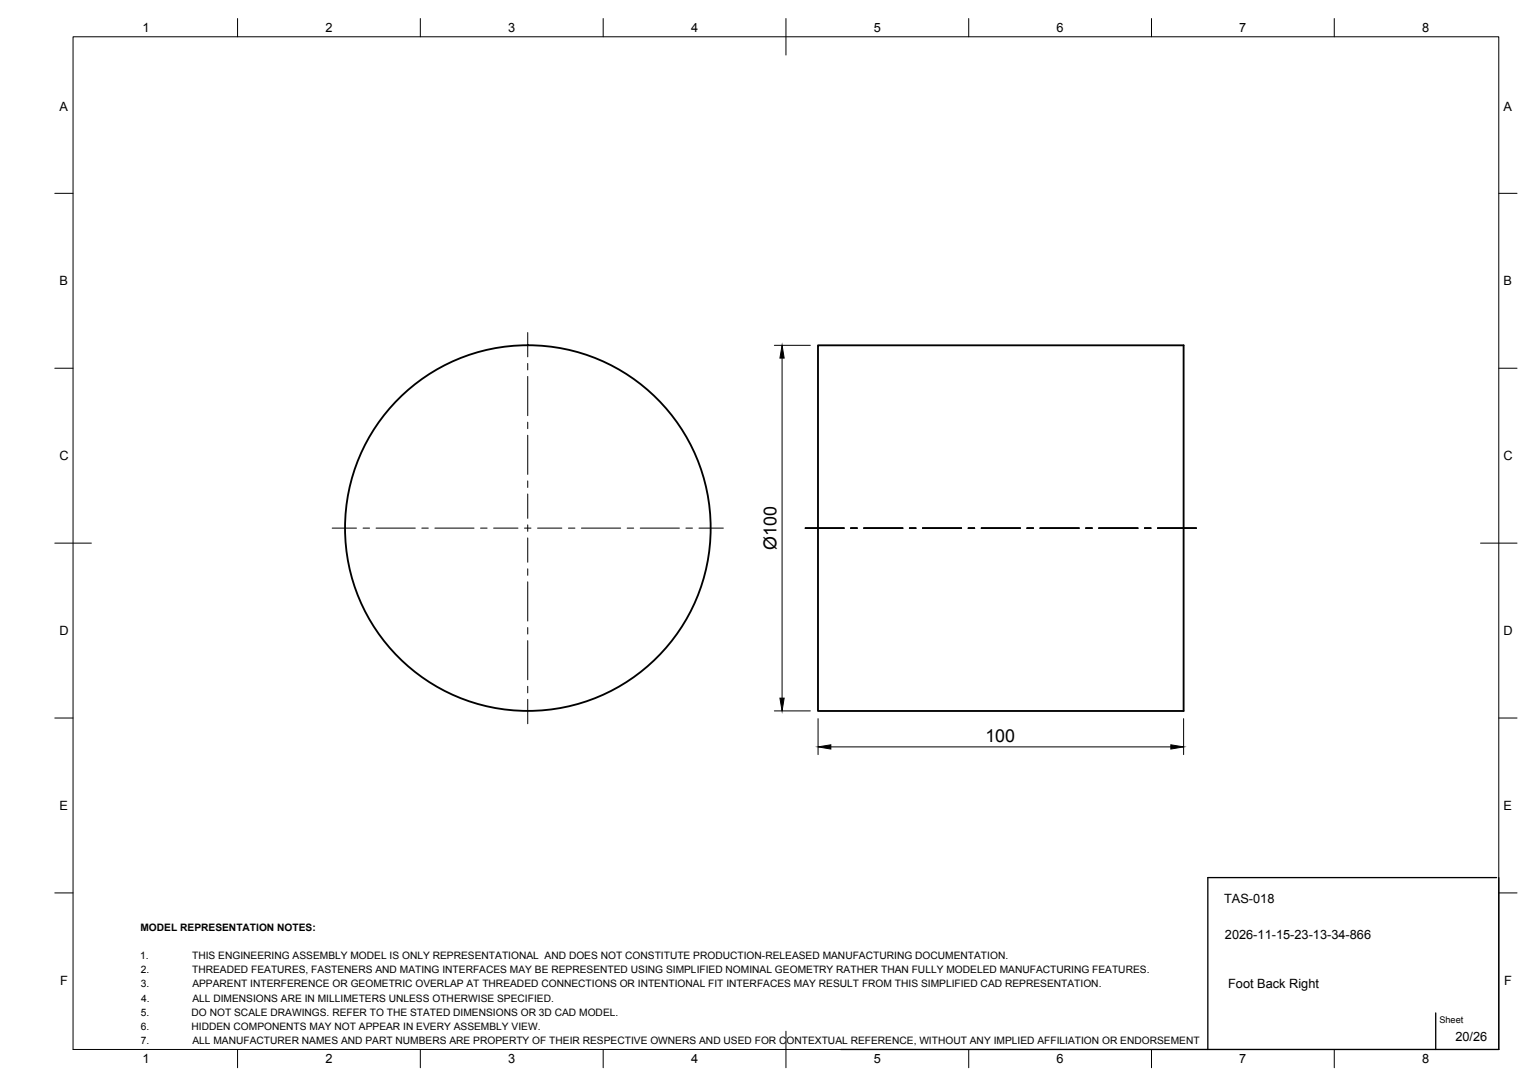
ISO-10303-21;
HEADER;
/* Generated by software containing ST-Developer
 * from STEP Tools, Inc. (www.steptools.com) 
 */

FILE_DESCRIPTION(
/* description */ (''),
/* implementation_level */ '2;1');

FILE_NAME(
/* name */ 'Foot Back Right.step',
/* time_stamp */ '2026-11-15T15:17:57-08:00',
/* author */ (''),
/* organization */ (''),
/* preprocessor_version */ 'ST-DEVELOPER v20.2',
/* originating_system */ 'Autodesk Translation Framework v15.17.0.0',
/* authorisation */ '');

FILE_SCHEMA (('AUTOMOTIVE_DESIGN { 1 0 10303 214 3 1 1 }'));
ENDSEC;

DATA;
#10=MECHANICAL_DESIGN_GEOMETRIC_PRESENTATION_REPRESENTATION('',(#195),#3723);
#17=CIRCLE('',#2442,1.96850393700787);
#18=CIRCLE('',#2443,1.96850393700787);
#26=CYLINDRICAL_SURFACE('',#2441,1.96850393700787);
#147=SHAPE_REPRESENTATION_RELATIONSHIP('SRR','None',#3828,#171);
#171=ADVANCED_BREP_SHAPE_REPRESENTATION('',(#219),#3717);
#195=STYLED_ITEM('',(#3945),#219);
#219=MANIFOLD_SOLID_BREP('Body1',#2043);
#324=FACE_OUTER_BOUND('',#450,.T.);
#325=FACE_OUTER_BOUND('',#451,.T.);
#326=FACE_OUTER_BOUND('',#452,.T.);
#450=EDGE_LOOP('',(#1689,#1690,#1691,#1692));
#451=EDGE_LOOP('',(#1693));
#452=EDGE_LOOP('',(#1694));
#660=LINE('',#3543,#882);
#882=VECTOR('',#2944,1.96850393700787);
#1047=VERTEX_POINT('',#3540);
#1048=VERTEX_POINT('',#3542);
#1266=EDGE_CURVE('',#1047,#1047,#17,.T.);
#1267=EDGE_CURVE('',#1047,#1048,#660,.T.);
#1268=EDGE_CURVE('',#1048,#1048,#18,.T.);
#1689=ORIENTED_EDGE('',*,*,#1266,.T.);
#1690=ORIENTED_EDGE('',*,*,#1267,.T.);
#1691=ORIENTED_EDGE('',*,*,#1268,.F.);
#1692=ORIENTED_EDGE('',*,*,#1267,.F.);
#1693=ORIENTED_EDGE('',*,*,#1268,.T.);
#1694=ORIENTED_EDGE('',*,*,#1266,.F.);
#1875=PLANE('',#2444);
#1876=PLANE('',#2445);
#1998=ADVANCED_FACE('',(#324),#26,.T.);
#1999=ADVANCED_FACE('',(#325),#1875,.T.);
#2000=ADVANCED_FACE('',(#326),#1876,.F.);
#2043=CLOSED_SHELL('',(#1998,#1999,#2000));
#2440=AXIS2_PLACEMENT_3D('',#3538,#2938,#2939);
#2441=AXIS2_PLACEMENT_3D('',#3539,#2940,#2941);
#2442=AXIS2_PLACEMENT_3D('',#3541,#2942,#2943);
#2443=AXIS2_PLACEMENT_3D('',#3544,#2945,#2946);
#2444=AXIS2_PLACEMENT_3D('',#3545,#2947,#2948);
#2445=AXIS2_PLACEMENT_3D('',#3546,#2949,#2950);
#2938=DIRECTION('axis',(0.,0.,1.));
#2939=DIRECTION('refdir',(1.,0.,0.));
#2940=DIRECTION('center_axis',(0.,1.,0.));
#2941=DIRECTION('ref_axis',(0.,0.,1.));
#2942=DIRECTION('center_axis',(0.,-1.,0.));
#2943=DIRECTION('ref_axis',(0.,0.,-1.));
#2944=DIRECTION('',(0.,-1.,0.));
#2945=DIRECTION('center_axis',(0.,-1.,0.));
#2946=DIRECTION('ref_axis',(0.,0.,-1.));
#2947=DIRECTION('center_axis',(0.,-1.,0.));
#2948=DIRECTION('ref_axis',(0.,0.,-1.));
#2949=DIRECTION('center_axis',(0.,-1.,0.));
#2950=DIRECTION('ref_axis',(0.,0.,-1.));
#3538=CARTESIAN_POINT('',(0.,0.,0.));
#3539=CARTESIAN_POINT('Origin',(33.6377952755906,-4.91732638859567E-15,
2.36220472440945));
#3540=CARTESIAN_POINT('',(33.6377952755906,3.93700787401574,0.393700787401574));
#3541=CARTESIAN_POINT('Origin',(33.6377952755906,3.93700787401574,2.36220472440945));
#3542=CARTESIAN_POINT('',(33.6377952755906,-4.91732638859567E-15,0.393700787401574));
#3543=CARTESIAN_POINT('',(33.6377952755906,-4.91732638859567E-15,0.393700787401574));
#3544=CARTESIAN_POINT('Origin',(33.6377952755906,-4.91732638859567E-15,
2.36220472440945));
#3545=CARTESIAN_POINT('Origin',(33.6377952755906,-4.91732638859567E-15,
2.36220472440945));
#3546=CARTESIAN_POINT('Origin',(33.6377952755906,3.93700787401574,2.36220472440945));
#3690=UNCERTAINTY_MEASURE_WITH_UNIT(LENGTH_MEASURE(0.000393700787401575),
#3725,'DISTANCE_ACCURACY_VALUE',
'Maximum model space distance between geometric entities at asserted c
onnectivities');
#3696=UNCERTAINTY_MEASURE_WITH_UNIT(LENGTH_MEASURE(0.000393700787401575),
#3725,'DISTANCE_ACCURACY_VALUE',
'Maximum model space distance between geometric entities at asserted c
onnectivities');
#3717=(
GEOMETRIC_REPRESENTATION_CONTEXT(3)
GLOBAL_UNCERTAINTY_ASSIGNED_CONTEXT((#3690))
GLOBAL_UNIT_ASSIGNED_CONTEXT((#3725,#3729,#3730))
REPRESENTATION_CONTEXT('','3D')
);
#3723=(
GEOMETRIC_REPRESENTATION_CONTEXT(3)
GLOBAL_UNCERTAINTY_ASSIGNED_CONTEXT((#3696))
GLOBAL_UNIT_ASSIGNED_CONTEXT((#3725,#3729,#3730))
REPRESENTATION_CONTEXT('','3D')
);
#3724=DIMENSIONAL_EXPONENTS(1.,0.,0.,0.,0.,0.,0.);
#3725=(
CONVERSION_BASED_UNIT('inch',#3728)
LENGTH_UNIT()
NAMED_UNIT(#3724)
);
#3726=(
LENGTH_UNIT()
NAMED_UNIT(*)
SI_UNIT(.MILLI.,.METRE.)
);
#3728=LENGTH_MEASURE_WITH_UNIT(LENGTH_MEASURE(25.4),#3726);
#3729=(
NAMED_UNIT(*)
PLANE_ANGLE_UNIT()
SI_UNIT($,.RADIAN.)
);
#3730=(
NAMED_UNIT(*)
SI_UNIT($,.STERADIAN.)
SOLID_ANGLE_UNIT()
);
#3751=SHAPE_DEFINITION_REPRESENTATION(#3778,#3828);
#3778=PRODUCT_DEFINITION_SHAPE('',$,#3855);
#3828=SHAPE_REPRESENTATION('',(#2440),#3717);
#3834=PRODUCT_DEFINITION_CONTEXT('part definition',#3914,'design');
#3855=PRODUCT_DEFINITION('2026-11-15-23-13-34-866','Foot Back Right',#3881,
#3834);
#3881=PRODUCT_DEFINITION_FORMATION('',$,#3936);
#3914=APPLICATION_CONTEXT(
'Core Data for Automotive Mechanical Design Process');
#3915=PRODUCT_CONTEXT('part definition',#3914,'mechanical');
#3936=PRODUCT('2026-11-15-23-13-34-866','Foot Back Right',$,(#3915));
#3945=PRESENTATION_STYLE_ASSIGNMENT((#3953));
#3953=SURFACE_STYLE_USAGE(.BOTH.,#3961);
#3961=SURFACE_SIDE_STYLE('',(#3969));
#3969=SURFACE_STYLE_FILL_AREA(#3977);
#3977=FILL_AREA_STYLE('Black',(#3985));
#3985=FILL_AREA_STYLE_COLOUR('Black',#3993);
#3993=COLOUR_RGB('Black',0.0784313725490196,0.0784313725490196,0.0784313725490196);
ENDSEC;
END-ISO-10303-21;
